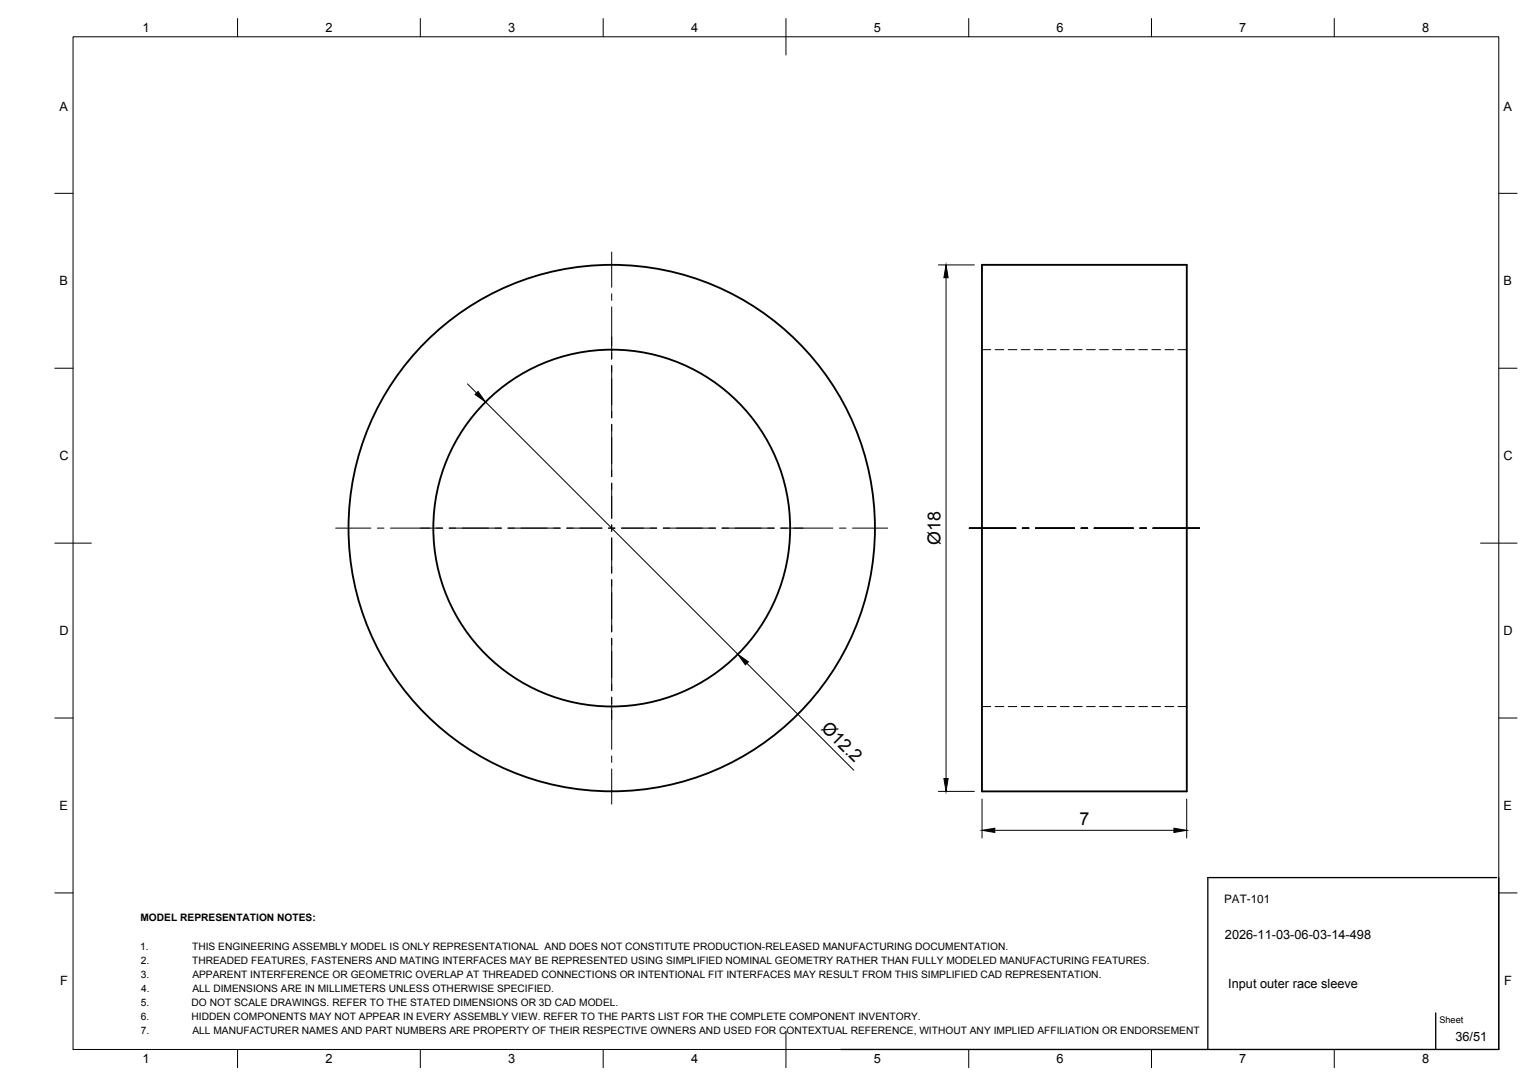
ISO-10303-21;
HEADER;
/* Generated by software containing ST-Developer
 * from STEP Tools, Inc. (www.steptools.com) 
 */

FILE_DESCRIPTION(
/* description */ ('Spur gear reduction stage 2-1 on bearing plates'),
/* implementation_level */ '2;1');

FILE_NAME(
/* name */ 'Input outer race sleeve.step',
/* time_stamp */ '2026-10-28T03:22:07-07:00',
/* author */ (''),
/* organization */ (''),
/* preprocessor_version */ 'ST-DEVELOPER v20.2',
/* originating_system */ 'Autodesk Translation Framework v15.17.0.0',
/* authorisation */ '');

FILE_SCHEMA (('AUTOMOTIVE_DESIGN { 1 0 10303 214 3 1 1 }'));
ENDSEC;

DATA;
#10=MECHANICAL_DESIGN_GEOMETRIC_PRESENTATION_REPRESENTATION('',(#990),#53909);
#889=SHAPE_REPRESENTATION_RELATIONSHIP('SRR','None',#54119,#932);
#932=ADVANCED_BREP_SHAPE_REPRESENTATION('',(#1045),#53893);
#990=STYLED_ITEM('',(#54397),#1045);
#1045=MANIFOLD_SOLID_BREP('Body1',#11317);
#1206=FACE_BOUND('',#2603,.T.);
#1207=FACE_BOUND('',#2605,.T.);
#1373=PLANE('',#12534);
#1374=PLANE('',#12535);
#1806=FACE_OUTER_BOUND('',#2600,.T.);
#1807=FACE_OUTER_BOUND('',#2601,.T.);
#1808=FACE_OUTER_BOUND('',#2602,.T.);
#1809=FACE_OUTER_BOUND('',#2604,.T.);
#2600=EDGE_LOOP('',(#8568,#8569,#8570,#8571));
#2601=EDGE_LOOP('',(#8572,#8573,#8574,#8575));
#2602=EDGE_LOOP('',(#8576));
#2603=EDGE_LOOP('',(#8577));
#2604=EDGE_LOOP('',(#8578));
#2605=EDGE_LOOP('',(#8579));
#3213=LINE('',#18076,#3854);
#3214=LINE('',#18082,#3855);
#3854=VECTOR('',#14666,0.61);
#3855=VECTOR('',#14673,0.9);
#4595=CIRCLE('',#12529,0.61);
#4596=CIRCLE('',#12530,0.61);
#4597=CIRCLE('',#12532,0.9);
#4598=CIRCLE('',#12533,0.9);
#5203=VERTEX_POINT('',#18073);
#5204=VERTEX_POINT('',#18075);
#5205=VERTEX_POINT('',#18079);
#5206=VERTEX_POINT('',#18081);
#6426=EDGE_CURVE('',#5203,#5203,#4595,.T.);
#6427=EDGE_CURVE('',#5203,#5204,#3213,.T.);
#6428=EDGE_CURVE('',#5204,#5204,#4596,.T.);
#6429=EDGE_CURVE('',#5205,#5205,#4597,.T.);
#6430=EDGE_CURVE('',#5205,#5206,#3214,.T.);
#6431=EDGE_CURVE('',#5206,#5206,#4598,.T.);
#8568=ORIENTED_EDGE('',*,*,#6426,.F.);
#8569=ORIENTED_EDGE('',*,*,#6427,.T.);
#8570=ORIENTED_EDGE('',*,*,#6428,.T.);
#8571=ORIENTED_EDGE('',*,*,#6427,.F.);
#8572=ORIENTED_EDGE('',*,*,#6429,.F.);
#8573=ORIENTED_EDGE('',*,*,#6430,.T.);
#8574=ORIENTED_EDGE('',*,*,#6431,.T.);
#8575=ORIENTED_EDGE('',*,*,#6430,.F.);
#8576=ORIENTED_EDGE('',*,*,#6429,.T.);
#8577=ORIENTED_EDGE('',*,*,#6426,.T.);
#8578=ORIENTED_EDGE('',*,*,#6431,.F.);
#8579=ORIENTED_EDGE('',*,*,#6428,.F.);
#10534=CYLINDRICAL_SURFACE('',#12528,0.61);
#10535=CYLINDRICAL_SURFACE('',#12531,0.9);
#10926=ADVANCED_FACE('',(#1806),#10534,.F.);
#10927=ADVANCED_FACE('',(#1807),#10535,.T.);
#10928=ADVANCED_FACE('',(#1808,#1206),#1373,.T.);
#10929=ADVANCED_FACE('',(#1809,#1207),#1374,.F.);
#11317=CLOSED_SHELL('',(#10926,#10927,#10928,#10929));
#12527=AXIS2_PLACEMENT_3D('',#18071,#14660,#14661);
#12528=AXIS2_PLACEMENT_3D('',#18072,#14662,#14663);
#12529=AXIS2_PLACEMENT_3D('',#18074,#14664,#14665);
#12530=AXIS2_PLACEMENT_3D('',#18077,#14667,#14668);
#12531=AXIS2_PLACEMENT_3D('',#18078,#14669,#14670);
#12532=AXIS2_PLACEMENT_3D('',#18080,#14671,#14672);
#12533=AXIS2_PLACEMENT_3D('',#18083,#14674,#14675);
#12534=AXIS2_PLACEMENT_3D('',#18084,#14676,#14677);
#12535=AXIS2_PLACEMENT_3D('',#18085,#14678,#14679);
#14660=DIRECTION('axis',(0.,0.,1.));
#14661=DIRECTION('refdir',(1.,0.,0.));
#14662=DIRECTION('center_axis',(0.,1.,0.));
#14663=DIRECTION('ref_axis',(1.,0.,0.));
#14664=DIRECTION('center_axis',(0.,-1.,0.));
#14665=DIRECTION('ref_axis',(1.,0.,0.));
#14666=DIRECTION('',(0.,-1.,0.));
#14667=DIRECTION('center_axis',(0.,-1.,0.));
#14668=DIRECTION('ref_axis',(1.,0.,0.));
#14669=DIRECTION('center_axis',(0.,1.,0.));
#14670=DIRECTION('ref_axis',(1.,0.,0.));
#14671=DIRECTION('center_axis',(0.,1.,0.));
#14672=DIRECTION('ref_axis',(1.,0.,0.));
#14673=DIRECTION('',(0.,-1.,0.));
#14674=DIRECTION('center_axis',(0.,1.,0.));
#14675=DIRECTION('ref_axis',(1.,0.,0.));
#14676=DIRECTION('center_axis',(0.,1.,0.));
#14677=DIRECTION('ref_axis',(1.,0.,0.));
#14678=DIRECTION('center_axis',(0.,1.,0.));
#14679=DIRECTION('ref_axis',(1.,0.,0.));
#18071=CARTESIAN_POINT('',(0.,0.,0.));
#18072=CARTESIAN_POINT('Origin',(0.,-4.7,0.));
#18073=CARTESIAN_POINT('',(-0.61,-4.,7.47034547479885E-17));
#18074=CARTESIAN_POINT('Origin',(0.,-4.,0.));
#18075=CARTESIAN_POINT('',(-0.61,-4.7,7.47034547479885E-17));
#18076=CARTESIAN_POINT('',(-0.61,-4.7,7.47034547479885E-17));
#18077=CARTESIAN_POINT('Origin',(0.,-4.7,0.));
#18078=CARTESIAN_POINT('Origin',(0.,-4.7,0.));
#18079=CARTESIAN_POINT('',(-0.9,-4.,1.10218211923262E-16));
#18080=CARTESIAN_POINT('Origin',(0.,-4.,0.));
#18081=CARTESIAN_POINT('',(-0.9,-4.7,1.10218211923262E-16));
#18082=CARTESIAN_POINT('',(-0.9,-4.7,1.10218211923262E-16));
#18083=CARTESIAN_POINT('Origin',(0.,-4.7,0.));
#18084=CARTESIAN_POINT('Origin',(0.,-4.,0.));
#18085=CARTESIAN_POINT('Origin',(0.,-4.7,0.));
#53843=UNCERTAINTY_MEASURE_WITH_UNIT(LENGTH_MEASURE(0.001),#53910,
'DISTANCE_ACCURACY_VALUE',
'Maximum model space distance between geometric entities at asserted c
onnectivities');
#53859=UNCERTAINTY_MEASURE_WITH_UNIT(LENGTH_MEASURE(0.001),#53910,
'DISTANCE_ACCURACY_VALUE',
'Maximum model space distance between geometric entities at asserted c
onnectivities');
#53893=(
GEOMETRIC_REPRESENTATION_CONTEXT(3)
GLOBAL_UNCERTAINTY_ASSIGNED_CONTEXT((#53843))
GLOBAL_UNIT_ASSIGNED_CONTEXT((#53910,#53912,#53913))
REPRESENTATION_CONTEXT('','3D')
);
#53909=(
GEOMETRIC_REPRESENTATION_CONTEXT(3)
GLOBAL_UNCERTAINTY_ASSIGNED_CONTEXT((#53859))
GLOBAL_UNIT_ASSIGNED_CONTEXT((#53910,#53912,#53913))
REPRESENTATION_CONTEXT('','3D')
);
#53910=(
LENGTH_UNIT()
NAMED_UNIT(*)
SI_UNIT(.CENTI.,.METRE.)
);
#53912=(
NAMED_UNIT(*)
PLANE_ANGLE_UNIT()
SI_UNIT($,.RADIAN.)
);
#53913=(
NAMED_UNIT(*)
SI_UNIT($,.STERADIAN.)
SOLID_ANGLE_UNIT()
);
#53947=SHAPE_DEFINITION_REPRESENTATION(#54045,#54119);
#54045=PRODUCT_DEFINITION_SHAPE('',$,#54169);
#54119=SHAPE_REPRESENTATION('',(#12527),#53893);
#54135=PRODUCT_DEFINITION_CONTEXT('part definition',#54284,'design');
#54169=PRODUCT_DEFINITION('Input outer race sleeve',
'Input outer race sleeve',#54218,#54135);
#54218=PRODUCT_DEFINITION_FORMATION('',$,#54319);
#54284=APPLICATION_CONTEXT(
'Core Data for Automotive Mechanical Design Process');
#54285=PRODUCT_CONTEXT('part definition',#54284,'mechanical');
#54319=PRODUCT('Input outer race sleeve','Input outer race sleeve',
'Input outer race sleeve',(#54285));
#54391=COLOUR_RGB('Grey',0.48,0.52,0.57);
#54392=FILL_AREA_STYLE_COLOUR('',#54391);
#54393=FILL_AREA_STYLE('',(#54392));
#54394=SURFACE_STYLE_FILL_AREA(#54393);
#54395=SURFACE_SIDE_STYLE('',(#54394));
#54396=SURFACE_STYLE_USAGE(.BOTH.,#54395);
#54397=PRESENTATION_STYLE_ASSIGNMENT((#54396));
ENDSEC;
END-ISO-10303-21;
